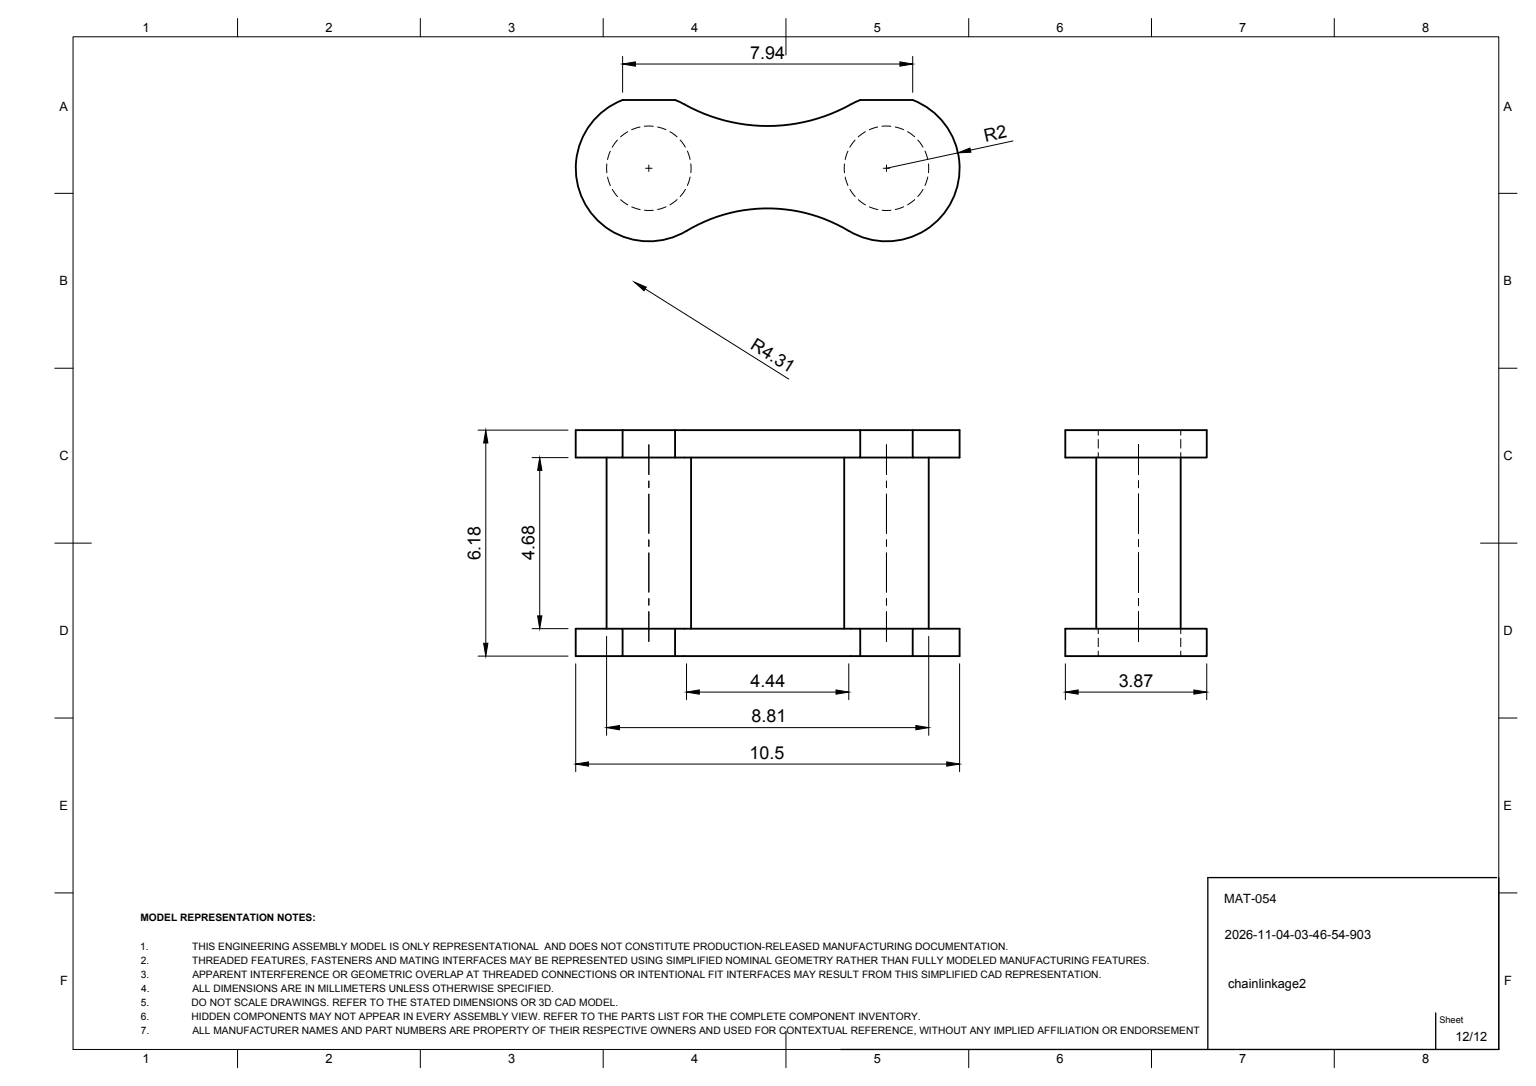
ISO-10303-21;
HEADER;
FILE_DESCRIPTION (('STEP AP214'),
    '1' );
FILE_NAME ('chainlinkage2.step',
    '2026-10-21T17:50:41',
    ( '' ),
    ( '' ),
    'SwSTEP 2.0',
    'SolidWorks 2026',
    '' );
FILE_SCHEMA (( 'AUTOMOTIVE_DESIGN' ));
ENDSEC;

DATA;
#33=CYLINDRICAL_SURFACE ( 'NONE', #30156, 1.999999999999999556 ) ;
#57=AXIS2_PLACEMENT_3D ( 'NONE', #27982, #32829, #17674 ) ;
#76=FACE_OUTER_BOUND ( 'NONE', #742, .T. ) ;
#123=DIRECTION ( 'NONE',  ( -0.000000000000000000, -0.000000000000000000, -1.000000000000000000 ) ) ;
#148=ORIENTED_EDGE ( 'NONE', *, *, #23576, .T. ) ;
#153=FACE_OUTER_BOUND ( 'NONE', #33687, .T. ) ;
#161=AXIS2_PLACEMENT_3D ( 'NONE', #27880, #20415, #25206 ) ;
#192=VERTEX_POINT ( 'NONE', #13936 ) ;
#226=CIRCLE ( 'NONE', #8162, 1.999999999999999112 ) ;
#270=ORIENTED_EDGE ( 'NONE', *, *, #32963, .T. ) ;
#279=CIRCLE ( 'NONE', #22435, 4.682234377621698584 ) ;
#283=CIRCLE ( 'NONE', #32662, 4.682234377621698584 ) ;
#306=DIRECTION ( 'NONE',  ( -0.000000000000000000, -0.000000000000000000, -1.000000000000000000 ) ) ;
#382=EDGE_CURVE ( 'NONE', #29286, #20322, #3767, .T. ) ;
#445=DIRECTION ( 'NONE',  ( 1.000000000000000000, 0.000000000000000000, 0.000000000000000000 ) ) ;
#472=CARTESIAN_POINT ( 'NONE',  ( -5.781867695661277118, -1.866624223957557893, -0.7500000000000000000 ) ) ;
#526=ORIENTED_EDGE ( 'NONE', *, *, #22218, .F. ) ;
#607=ORIENTED_EDGE ( 'NONE', *, *, #23373, .T. ) ;
#610=EDGE_CURVE ( 'NONE', #19346, #10620, #34542, .T. ) ;
#657=EDGE_CURVE ( 'NONE', #30105, #32001, #24381, .T. ) ;
#669=DIRECTION ( 'NONE',  ( -1.000000000000000000, 0.000000000000000000, 0.000000000000000000 ) ) ;
#680=ORIENTED_EDGE ( 'NONE', *, *, #6279, .T. ) ;
#740=CARTESIAN_POINT ( 'NONE',  ( -8.499999999999998224, 0.000000000000000000, 5.429999999999999716 ) ) ;
#742=EDGE_LOOP ( 'NONE', ( #25177, #23804, #31066, #16632 ) ) ;
#807=ORIENTED_EDGE ( 'NONE', *, *, #3982, .T. ) ;
#962=AXIS2_PLACEMENT_3D ( 'NONE', #16567, #5499, #19235 ) ;
#981=CARTESIAN_POINT ( 'NONE',  ( -0.9727285265192158192, -1.747512292859697114, 5.429999999999999716 ) ) ;
#994=ORIENTED_EDGE ( 'NONE', *, *, #20204, .T. ) ;
#1062=AXIS2_PLACEMENT_3D ( 'NONE', #28487, #22452, #19618 ) ;
#1071=CARTESIAN_POINT ( 'NONE',  ( -7.218132304338721994, -1.866624223957557893, -0.7500000000000000000 ) ) ;
#1096=AXIS2_PLACEMENT_3D ( 'NONE', #14859, #9508, #17884 ) ;
#1169=CARTESIAN_POINT ( 'NONE',  ( -0.7181323043387224381, -1.866624223957557893, 5.429999999999999716 ) ) ;
#1232=VECTOR ( 'NONE', #14059, 1000.000000000000000 ) ;
#1326=CARTESIAN_POINT ( 'NONE',  ( -6.500000000000000000, 0.000000000000000000, 4.679999999999999716 ) ) ;
#1403=ADVANCED_FACE ( 'NONE', ( #7003 ), #23561, .T. ) ;
#1433=CARTESIAN_POINT ( 'NONE',  ( -6.500000000000000000, 0.000000000000000000, -0.7500000000000000000 ) ) ;
#1457=DIRECTION ( 'NONE',  ( 1.000000000000000000, 0.000000000000000000, 0.000000000000000000 ) ) ;
#1552=ORIENTED_EDGE ( 'NONE', *, *, #6009, .F. ) ;
#1599=EDGE_CURVE ( 'NONE', #27420, #3383, #29381, .T. ) ;
#1635=EDGE_CURVE ( 'NONE', #15525, #19610, #9424, .T. ) ;
#1664=DIRECTION ( 'NONE',  ( 1.000000000000000000, 0.000000000000000000, -0.000000000000000000 ) ) ;
#1772=CARTESIAN_POINT ( 'NONE',  ( -5.527271473480783293, -1.747512292859696226, -0.7500000000000000000 ) ) ;
#1795=DIRECTION ( 'NONE',  ( -0.000000000000000000, -0.000000000000000000, 1.000000000000000000 ) ) ;
#1801=VERTEX_POINT ( 'NONE', #11106 ) ;
#1824=ORIENTED_EDGE ( 'NONE', *, *, #20677, .F. ) ;
#1889=EDGE_CURVE ( 'NONE', #30258, #28753, #22427, .T. ) ;
#1906=ORIENTED_EDGE ( 'NONE', *, *, #14574, .T. ) ;
#1963=DIRECTION ( 'NONE',  ( 0.000000000000000000, 0.000000000000000000, 1.000000000000000000 ) ) ;
#2042=ORIENTED_EDGE ( 'NONE', *, *, #610, .T. ) ;
#2140=FACE_OUTER_BOUND ( 'NONE', #7438, .T. ) ;
#2145=EDGE_CURVE ( 'NONE', #12065, #19610, #21352, .T. ) ;
#2200=DIRECTION ( 'NONE',  ( 0.000000000000000000, 0.000000000000000000, 1.000000000000000000 ) ) ;
#2218=DIRECTION ( 'NONE',  ( -0.000000000000000000, -0.000000000000000000, 1.000000000000000000 ) ) ;
#2279=CYLINDRICAL_SURFACE ( 'NONE', #5773, 4.306175033202026547 ) ;
#2373=CARTESIAN_POINT ( 'NONE',  ( -3.250000000000000000, -5.838643359331793015, 0.000000000000000000 ) ) ;
#2446=EDGE_LOOP ( 'NONE', ( #12551, #26713, #15573, #807 ) ) ;
#2510=CARTESIAN_POINT ( 'NONE',  ( -0.9727285265192158192, -1.747512292859697114, 5.429999999999999716 ) ) ;
#2547=EDGE_LOOP ( 'NONE', ( #27809, #20644, #34283, #22240 ) ) ;
#2562=EDGE_CURVE ( 'NONE', #24130, #18561, #30361, .T. ) ;
#2601=DIRECTION ( 'NONE',  ( -0.000000000000000000, -0.000000000000000000, 1.000000000000000000 ) ) ;
#2706=DIRECTION ( 'NONE',  ( 0.000000000000000000, 0.000000000000000000, 1.000000000000000000 ) ) ;
#2718=EDGE_CURVE ( 'NONE', #20895, #32553, #27626, .T. ) ;
#2738=LINE ( 'NONE', #10594, #16975 ) ;
#2747=CARTESIAN_POINT ( 'NONE',  ( -8.499999999999998224, 0.000000000000000000, 5.429999999999999716 ) ) ;
#2801=CARTESIAN_POINT ( 'NONE',  ( -5.781867695661277118, -1.866624223957557671, 0.000000000000000000 ) ) ;
#2898=AXIS2_PLACEMENT_3D ( 'NONE', #17177, #17360, #3961 ) ;
#2943=ORIENTED_EDGE ( 'NONE', *, *, #23576, .F. ) ;
#3000=LINE ( 'NONE', #33080, #33940 ) ;
#3027=EDGE_LOOP ( 'NONE', ( #24950, #28921 ) ) ;
#3202=EDGE_CURVE ( 'NONE', #20895, #30258, #14676, .T. ) ;
#3264=ORIENTED_EDGE ( 'NONE', *, *, #15668, .T. ) ;
#3331=CYLINDRICAL_SURFACE ( 'NONE', #18823, 1.999999999999999556 ) ;
#3383=VERTEX_POINT ( 'NONE', #7675 ) ;
#3421=EDGE_LOOP ( 'NONE', ( #14691, #9777, #5394, #24495 ) ) ;
#3565=FACE_OUTER_BOUND ( 'NONE', #34074, .T. ) ;
#3575=DIRECTION ( 'NONE',  ( -0.000000000000000000, -0.000000000000000000, 1.000000000000000000 ) ) ;
#3586=CARTESIAN_POINT ( 'NONE',  ( -6.500000000000000000, 0.000000000000000000, 5.429999999999999716 ) ) ;
#3600=DIRECTION ( 'NONE',  ( 0.000000000000000000, 0.000000000000000000, -1.000000000000000000 ) ) ;
#3637=EDGE_LOOP ( 'NONE', ( #26902, #13289, #29468, #6440 ) ) ;
#3645=AXIS2_PLACEMENT_3D ( 'NONE', #27958, #9269, #24755 ) ;
#3673=EDGE_LOOP ( 'NONE', ( #24652, #23698 ) ) ;
#3680=EDGE_CURVE ( 'NONE', #29286, #8432, #26053, .T. ) ;
#3707=LINE ( 'NONE', #11740, #27308 ) ;
#3708=ORIENTED_EDGE ( 'NONE', *, *, #1599, .F. ) ;
#3740=ORIENTED_EDGE ( 'NONE', *, *, #1599, .T. ) ;
#3752=AXIS2_PLACEMENT_3D ( 'NONE', #13925, #19628, #2706 ) ;
#3767=LINE ( 'NONE', #22120, #5990 ) ;
#3899=VECTOR ( 'NONE', #5620, 1000.000000000000000 ) ;
#3961=DIRECTION ( 'NONE',  ( -1.000000000000000000, 0.000000000000000000, 0.000000000000000000 ) ) ;
#3982=EDGE_CURVE ( 'NONE', #28753, #32553, #7816, .T. ) ;
#3987=ORIENTED_EDGE ( 'NONE', *, *, #33054, .F. ) ;
#4008=CIRCLE ( 'NONE', #57, 1.154999999999999805 ) ;
#4040=CARTESIAN_POINT ( 'NONE',  ( -6.500000000000000000, 0.000000000000000000, 5.429999999999999716 ) ) ;
#4043=DIRECTION ( 'NONE',  ( -0.000000000000000000, -0.000000000000000000, 1.000000000000000000 ) ) ;
#4060=DIRECTION ( 'NONE',  ( -1.000000000000000000, 0.000000000000000000, 0.000000000000000000 ) ) ;
#4081=DIRECTION ( 'NONE',  ( 0.000000000000000000, 0.000000000000000000, 1.000000000000000000 ) ) ;
#4084=ORIENTED_EDGE ( 'NONE', *, *, #2562, .F. ) ;
#4105=DIRECTION ( 'NONE',  ( -0.000000000000000000, -0.000000000000000000, -1.000000000000000000 ) ) ;
#4153=DIRECTION ( 'NONE',  ( -0.000000000000000000, -0.000000000000000000, 1.000000000000000000 ) ) ;
#4248=EDGE_LOOP ( 'NONE', ( #3740, #27735, #10056, #18991 ) ) ;
#4252=EDGE_CURVE ( 'NONE', #20322, #28753, #7368, .T. ) ;
#4270=ORIENTED_EDGE ( 'NONE', *, *, #32781, .T. ) ;
#4272=PLANE ( 'NONE',  #13542 ) ;
#4320=CARTESIAN_POINT ( 'NONE',  ( -1.625000000000000000, 2.702098422956710877, 4.679999999999999716 ) ) ;
#4327=CARTESIAN_POINT ( 'NONE',  ( -3.250000000000000000, 5.404196845913421754, -0.7500000000000000000 ) ) ;
#4356=ADVANCED_FACE ( 'NONE', ( #76 ), #10938, .T. ) ;
#4360=VERTEX_POINT ( 'NONE', #6274 ) ;
#4475=DIRECTION ( 'NONE',  ( -0.000000000000000000, -0.000000000000000000, -1.000000000000000000 ) ) ;
#4484=VECTOR ( 'NONE', #15412, 1000.000000000000000 ) ;
#4561=EDGE_CURVE ( 'NONE', #32547, #7170, #25532, .T. ) ;
#4648=CARTESIAN_POINT ( 'NONE',  ( -0.7181323043387224381, -1.866624223957557893, -0.7500000000000000000 ) ) ;
#4699=LINE ( 'NONE', #2747, #20213 ) ;
#4788=EDGE_CURVE ( 'NONE', #25489, #15525, #27437, .T. ) ;
#4841=APPLICATION_CONTEXT ( 'automotive_design' ) ;
#4877=CIRCLE ( 'NONE', #28201, 1.154999999999999805 ) ;
#4907=AXIS2_PLACEMENT_3D ( 'NONE', #20412, #12059, #23256 ) ;
#5009=LINE ( 'NONE', #24050, #23783 ) ;
#5104=CARTESIAN_POINT ( 'NONE',  ( -5.781867695661277118, -1.866624223957557671, 4.679999999999999716 ) ) ;
#5132=DIRECTION ( 'NONE',  ( 1.000000000000000000, 0.000000000000000000, 0.000000000000000000 ) ) ;
#5180=FACE_OUTER_BOUND ( 'NONE', #20182, .T. ) ;
#5206=EDGE_CURVE ( 'NONE', #24311, #10245, #32875, .T. ) ;
#5210=ORIENTED_EDGE ( 'NONE', *, *, #34210, .F. ) ;
#5394=ORIENTED_EDGE ( 'NONE', *, *, #14375, .T. ) ;
#5415=DIRECTION ( 'NONE',  ( 1.000000000000000000, 0.000000000000000000, 0.000000000000000000 ) ) ;
#5431=ORIENTED_EDGE ( 'NONE', *, *, #19622, .T. ) ;
#5455=LINE ( 'NONE', #13653, #3899 ) ;
#5456=ORIENTED_EDGE ( 'NONE', *, *, #15677, .F. ) ;
#5499=DIRECTION ( 'NONE',  ( 0.000000000000000000, 0.000000000000000000, -1.000000000000000000 ) ) ;
#5531=DIRECTION ( 'NONE',  ( -0.000000000000000000, -0.000000000000000000, -1.000000000000000000 ) ) ;
#5620=DIRECTION ( 'NONE',  ( 1.000000000000000000, -0.000000000000000000, -0.000000000000000000 ) ) ;
#5648=VECTOR ( 'NONE', #5531, 1000.000000000000000 ) ;
#5753=CYLINDRICAL_SURFACE ( 'NONE', #12901, 1.999999999999999556 ) ;
#5773=AXIS2_PLACEMENT_3D ( 'NONE', #10296, #13502, #24337 ) ;
#5812=ADVANCED_FACE ( 'NONE', ( #3565 ), #22273, .T. ) ;
#5894=( NAMED_UNIT ( * ) SI_UNIT ( $, .STERADIAN. ) SOLID_ANGLE_UNIT ( ) );
#5905=CIRCLE ( 'NONE', #29220, 1.155000000000000027 ) ;
#5962=CARTESIAN_POINT ( 'NONE',  ( -7.218132304338721994, -1.866624223957557893, 5.429999999999999716 ) ) ;
#5972=DIRECTION ( 'NONE',  ( -1.000000000000000000, 0.000000000000000000, 0.000000000000000000 ) ) ;
#5990=VECTOR ( 'NONE', #8937, 1000.000000000000000 ) ;
#6009=EDGE_CURVE ( 'NONE', #10891, #18561, #14477, .T. ) ;
#6062=ORIENTED_EDGE ( 'NONE', *, *, #32625, .F. ) ;
#6080=EDGE_CURVE ( 'NONE', #14482, #29522, #13328, .T. ) ;
#6147=CARTESIAN_POINT ( 'NONE',  ( 0.7181323043387221050, -1.866624223957557893, -0.7500000000000000000 ) ) ;
#6183=ORIENTED_EDGE ( 'NONE', *, *, #382, .F. ) ;
#6198=ORIENTED_EDGE ( 'NONE', *, *, #657, .F. ) ;
#6223=CARTESIAN_POINT ( 'NONE',  ( 0.000000000000000000, 0.000000000000000000, -0.7500000000000000000 ) ) ;
#6274=CARTESIAN_POINT ( 'NONE',  ( -5.781867695661277118, -1.866624223957557893, 5.429999999999999716 ) ) ;
#6276=CARTESIAN_POINT ( 'NONE',  ( 2.630124765083918348, -1.866624223957557893, 5.429999999999999716 ) ) ;
#6279=EDGE_CURVE ( 'NONE', #8432, #10891, #283, .T. ) ;
#6364=ORIENTED_EDGE ( 'NONE', *, *, #22218, .T. ) ;
#6440=ORIENTED_EDGE ( 'NONE', *, *, #12810, .T. ) ;
#6484=ORIENTED_EDGE ( 'NONE', *, *, #28737, .F. ) ;
#6499=ORIENTED_EDGE ( 'NONE', *, *, #23373, .F. ) ;
#6540=PLANE ( 'NONE',  #23252 ) ;
#6625=AXIS2_PLACEMENT_3D ( 'NONE', #7346, #10210, #28729 ) ;
#6650=ADVANCED_FACE ( 'NONE', ( #32164 ), #13134, .T. ) ;
#6750=AXIS2_PLACEMENT_3D ( 'NONE', #22899, #25556, #33751 ) ;
#6774=DIRECTION ( 'NONE',  ( 0.000000000000000000, 1.000000000000000000, -0.000000000000000000 ) ) ;
#6790=( LENGTH_UNIT ( ) NAMED_UNIT ( * ) SI_UNIT ( .MILLI., .METRE. ) );
#6808=DIRECTION ( 'NONE',  ( -1.000000000000000000, 0.000000000000000000, 0.000000000000000000 ) ) ;
#6821=DIRECTION ( 'NONE',  ( -0.000000000000000000, -0.000000000000000000, -1.000000000000000000 ) ) ;
#6836=VERTEX_POINT ( 'NONE', #33564 ) ;
#6850=DIRECTION ( 'NONE',  ( 1.000000000000000000, 0.000000000000000000, 0.000000000000000000 ) ) ;
#6866=CARTESIAN_POINT ( 'NONE',  ( -3.250000000000000000, 5.404196845913421754, 5.429999999999999716 ) ) ;
#6941=CARTESIAN_POINT ( 'NONE',  ( 2.630124765083918348, -1.866624223957557893, 5.429999999999999716 ) ) ;
#6960=( NAMED_UNIT ( * ) SI_UNIT ( $, .STERADIAN. ) SOLID_ANGLE_UNIT ( ) );
#7003=FACE_OUTER_BOUND ( 'NONE', #3637, .T. ) ;
#7012=DIRECTION ( 'NONE',  ( 1.000000000000000000, 0.000000000000000000, 0.000000000000000000 ) ) ;
#7051=VECTOR ( 'NONE', #1795, 1000.000000000000000 ) ;
#7067=CARTESIAN_POINT ( 'NONE',  ( -6.500000000000000000, 0.000000000000000000, 0.000000000000000000 ) ) ;
#7073=VERTEX_POINT ( 'NONE', #7914 ) ;
#7107=CARTESIAN_POINT ( 'NONE',  ( -6.500000000000000000, 0.000000000000000000, 5.429999999999999716 ) ) ;
#7145=DIRECTION ( 'NONE',  ( 0.000000000000000000, 0.000000000000000000, 1.000000000000000000 ) ) ;
#7170=VERTEX_POINT ( 'NONE', #22325 ) ;
#7205=CARTESIAN_POINT ( 'NONE',  ( -5.527271473480783293, -1.747512292859696226, 5.429999999999999716 ) ) ;
#7230=CARTESIAN_POINT ( 'NONE',  ( -1.030735741678193484, 1.713938105891546826, 0.000000000000000000 ) ) ;
#7325=DIRECTION ( 'NONE',  ( 0.000000000000000000, 0.000000000000000000, 1.000000000000000000 ) ) ;
#7346=CARTESIAN_POINT ( 'NONE',  ( 0.000000000000000000, 0.000000000000000000, 4.679999999999999716 ) ) ;
#7368=LINE ( 'NONE', #34983, #4484 ) ;
#7438=EDGE_LOOP ( 'NONE', ( #13903, #20764, #6198, #1824 ) ) ;
#7472=DIRECTION ( 'NONE',  ( 0.000000000000000000, 0.000000000000000000, 1.000000000000000000 ) ) ;
#7500=EDGE_LOOP ( 'NONE', ( #17353, #22619, #28907, #19252 ) ) ;
#7618=ADVANCED_FACE ( 'NONE', ( #16787 ), #21583, .F. ) ;
#7628=DIRECTION ( 'NONE',  ( -0.000000000000000000, -0.000000000000000000, -1.000000000000000000 ) ) ;
#7675=CARTESIAN_POINT ( 'NONE',  ( -5.527271473480783293, -1.747512292859696226, 0.000000000000000000 ) ) ;
#7677=ORIENTED_EDGE ( 'NONE', *, *, #1635, .T. ) ;
#7816=LINE ( 'NONE', #6147, #34613 ) ;
#7914=CARTESIAN_POINT ( 'NONE',  ( -5.469264258321805627, 1.713938105891546382, -0.7500000000000000000 ) ) ;
#7930=DIRECTION ( 'NONE',  ( 0.000000000000000000, 0.000000000000000000, 1.000000000000000000 ) ) ;
#7953=CARTESIAN_POINT ( 'NONE',  ( -5.781867695661277118, -1.866624223957557893, 5.429999999999999716 ) ) ;
#7982=AXIS2_PLACEMENT_3D ( 'NONE', #19006, #123, #5972 ) ;
#8095=ORIENTED_EDGE ( 'NONE', *, *, #9484, .F. ) ;
#8124=( GEOMETRIC_REPRESENTATION_CONTEXT ( 3 ) GLOBAL_UNCERTAINTY_ASSIGNED_CONTEXT ( ( #10711 ) ) GLOBAL_UNIT_ASSIGNED_CONTEXT ( ( #6790, #17854, #6960 ) ) REPRESENTATION_CONTEXT ( 'NONE', 'WORKASPACE' ) );
#8162=AXIS2_PLACEMENT_3D ( 'NONE', #16370, #27200, #18690 ) ;
#8188=ADVANCED_FACE ( 'NONE', ( #31428 ), #12407, .T. ) ;
#8209=ORIENTED_EDGE ( 'NONE', *, *, #20677, .T. ) ;
#8237=EDGE_CURVE ( 'NONE', #25058, #192, #14735, .T. ) ;
#8298=DIRECTION ( 'NONE',  ( -1.000000000000000000, 0.000000000000000000, 0.000000000000000000 ) ) ;
#8328=VECTOR ( 'NONE', #23417, 1000.000000000000000 ) ;
#8350=EDGE_CURVE ( 'NONE', #29522, #33375, #4699, .T. ) ;
#8432=VERTEX_POINT ( 'NONE', #21094 ) ;
#8444=ADVANCED_FACE ( 'NONE', ( #19148 ), #5753, .T. ) ;
#8460=ORIENTED_EDGE ( 'NONE', *, *, #17006, .F. ) ;
#8549=ORIENTED_EDGE ( 'NONE', *, *, #14574, .F. ) ;
#8594=VECTOR ( 'NONE', #28010, 1000.000000000000000 ) ;
#8684=FACE_OUTER_BOUND ( 'NONE', #19828, .T. ) ;
#8792=CIRCLE ( 'NONE', #25839, 1.999999999999999112 ) ;
#8812=FACE_BOUND ( 'NONE', #3673, .T. ) ;
#8822=DIRECTION ( 'NONE',  ( 0.000000000000000000, 0.000000000000000000, -1.000000000000000000 ) ) ;
#8913=DIRECTION ( 'NONE',  ( 1.000000000000000000, 0.000000000000000000, 0.000000000000000000 ) ) ;
#8937=DIRECTION ( 'NONE',  ( -0.000000000000000000, -0.000000000000000000, 1.000000000000000000 ) ) ;
#8941=CARTESIAN_POINT ( 'NONE',  ( -1.155000000000000027, 0.000000000000000000, 4.679999999999999716 ) ) ;
#8944=LINE ( 'NONE', #19816, #15535 ) ;
#9132=CARTESIAN_POINT ( 'NONE',  ( -6.500000000000000000, 0.000000000000000000, 4.679999999999999716 ) ) ;
#9140=AXIS2_PLACEMENT_3D ( 'NONE', #25229, #13124, #10266 ) ;
#9166=VERTEX_POINT ( 'NONE', #13020 ) ;
#9191=ORIENTED_EDGE ( 'NONE', *, *, #17768, .T. ) ;
#9269=DIRECTION ( 'NONE',  ( -0.000000000000000000, -0.000000000000000000, 1.000000000000000000 ) ) ;
#9292=EDGE_CURVE ( 'NONE', #26696, #10620, #16968, .T. ) ;
#9307=CARTESIAN_POINT ( 'NONE',  ( 0.000000000000000000, 0.000000000000000000, 0.000000000000000000 ) ) ;
#9356=AXIS2_PLACEMENT_3D ( 'NONE', #7107, #4081, #14977 ) ;
#9424=CIRCLE ( 'NONE', #32699, 1.999999999999999556 ) ;
#9484=EDGE_CURVE ( 'NONE', #15525, #19346, #14950, .T. ) ;
#9508=DIRECTION ( 'NONE',  ( -0.000000000000000000, -0.000000000000000000, -1.000000000000000000 ) ) ;
#9509=EDGE_LOOP ( 'NONE', ( #3264, #2042, #19117, #17931 ) ) ;
#9514=DIRECTION ( 'NONE',  ( 0.000000000000000000, 0.000000000000000000, 1.000000000000000000 ) ) ;
#9533=EDGE_CURVE ( 'NONE', #31862, #9166, #17099, .T. ) ;
#9557=ORIENTED_EDGE ( 'NONE', *, *, #17768, .F. ) ;
#9777=ORIENTED_EDGE ( 'NONE', *, *, #28737, .T. ) ;
#10056=ORIENTED_EDGE ( 'NONE', *, *, #6279, .F. ) ;
#10119=ADVANCED_FACE ( 'NONE', ( #153 ), #26678, .T. ) ;
#10166=ADVANCED_FACE ( 'NONE', ( #8684 ), #6540, .F. ) ;
#10191=CARTESIAN_POINT ( 'NONE',  ( -6.500000000000000000, 0.000000000000000000, 5.429999999999999716 ) ) ;
#10210=DIRECTION ( 'NONE',  ( -0.000000000000000000, -0.000000000000000000, -1.000000000000000000 ) ) ;
#10245=VERTEX_POINT ( 'NONE', #7230 ) ;
#10266=DIRECTION ( 'NONE',  ( -1.000000000000000000, 0.000000000000000000, 0.000000000000000000 ) ) ;
#10296=CARTESIAN_POINT ( 'NONE',  ( -3.250000000000000000, 5.404196845913421754, -0.7500000000000000000 ) ) ;
#10368=CARTESIAN_POINT ( 'NONE',  ( 1.999999999999999556, 0.000000000000000000, -0.7500000000000000000 ) ) ;
#10410=MECHANICAL_DESIGN_GEOMETRIC_PRESENTATION_REPRESENTATION('',(#34291),#14976);
#10424=CARTESIAN_POINT ( 'NONE',  ( -7.654999999999999361, 1.414467053015192657E-16, 0.000000000000000000 ) ) ;
#10486=EDGE_CURVE ( 'NONE', #32001, #1801, #22005, .T. ) ;
#10493=CARTESIAN_POINT ( 'NONE',  ( -6.500000000000000000, 0.000000000000000000, -0.7500000000000000000 ) ) ;
#10594=CARTESIAN_POINT ( 'NONE',  ( -5.344999999999999751, 0.000000000000000000, -0.7520000000000001128 ) ) ;
#10601=ORIENTED_EDGE ( 'NONE', *, *, #4788, .F. ) ;
#10603=DIRECTION ( 'NONE',  ( -0.000000000000000000, -0.000000000000000000, -1.000000000000000000 ) ) ;
#10620=VERTEX_POINT ( 'NONE', #1169 ) ;
#10656=ORIENTED_EDGE ( 'NONE', *, *, #15964, .F. ) ;
#10662=ORIENTED_EDGE ( 'NONE', *, *, #6080, .F. ) ;
#10700=EDGE_CURVE ( 'NONE', #7073, #24311, #14887, .T. ) ;
#10709=ORIENTED_EDGE ( 'NONE', *, *, #8350, .F. ) ;
#10711=UNCERTAINTY_MEASURE_WITH_UNIT (LENGTH_MEASURE( 1.000000000000000082E-05 ), #6790, 'distance_accuracy_value', 'NONE');
#10748=AXIS2_PLACEMENT_3D ( 'NONE', #10493, #21351, #22219 ) ;
#10774=EDGE_CURVE ( 'NONE', #26696, #12145, #24396, .T. ) ;
#10791=DIRECTION ( 'NONE',  ( 1.000000000000000000, 0.000000000000000000, 0.000000000000000000 ) ) ;
#10825=ADVANCED_FACE ( 'NONE', ( #14974 ), #32408, .T. ) ;
#10826=CARTESIAN_POINT ( 'NONE',  ( -4.875000000000000000, 2.702098422956710877, 0.000000000000000000 ) ) ;
#10854=LINE ( 'NONE', #32734, #1232 ) ;
#10867=DIRECTION ( 'NONE',  ( -1.000000000000000000, 0.000000000000000000, 0.000000000000000000 ) ) ;
#10887=DIRECTION ( 'NONE',  ( -0.000000000000000000, -0.000000000000000000, -1.000000000000000000 ) ) ;
#10891=VERTEX_POINT ( 'NONE', #1772 ) ;
#10938=CYLINDRICAL_SURFACE ( 'NONE', #15316, 1.999999999999999112 ) ;
#10944=DIRECTION ( 'NONE',  ( -0.000000000000000000, -0.000000000000000000, 1.000000000000000000 ) ) ;
#10974=VERTEX_POINT ( 'NONE', #33997 ) ;
#11099=CLOSED_SHELL ( 'NONE', ( #21470, #4356, #8444, #6650, #25183, #8188, #29310, #19441, #1403, #34762, #10825, #23574, #10119, #21762, #26582, #23268, #15805, #23565, #13258, #15277, #25660, #5812, #21609, #13668, #10166, #7618 ) ) ;
#11106=CARTESIAN_POINT ( 'NONE',  ( -7.218132304338721994, -1.866624223957557893, 5.429999999999999716 ) ) ;
#11108=ORIENTED_EDGE ( 'NONE', *, *, #32781, .F. ) ;
#11136=EDGE_CURVE ( 'NONE', #25489, #12065, #16989, .T. ) ;
#11168=CYLINDRICAL_SURFACE ( 'NONE', #7982, 4.306175033202026547 ) ;
#11202=PRODUCT ( 'chainlinkage2', 'chainlinkage2', '', ( #13725 ) ) ;
#11219=VECTOR ( 'NONE', #8822, 1000.000000000000000 ) ;
#11416=EDGE_LOOP ( 'NONE', ( #10709, #10662, #6364, #24149 ) ) ;
#11435=CARTESIAN_POINT ( 'NONE',  ( 0.7181323043387224381, -1.866624223957557893, -0.7500000000000000000 ) ) ;
#11453=CARTESIAN_POINT ( 'NONE',  ( -5.344999999999999751, 0.000000000000000000, 4.679999999999999716 ) ) ;
#11454=AXIS2_PLACEMENT_3D ( 'NONE', #31541, #7145, #25676 ) ;
#11481=CARTESIAN_POINT ( 'NONE',  ( 0.7181323043387224381, -1.866624223957557893, 5.429999999999999716 ) ) ;
#11525=ORIENTED_EDGE ( 'NONE', *, *, #3680, .T. ) ;
#11634=VECTOR ( 'NONE', #7628, 1000.000000000000000 ) ;
#11740=CARTESIAN_POINT ( 'NONE',  ( -7.218132304338721994, -1.866624223957557893, -0.7500000000000000000 ) ) ;
#11795=DIRECTION ( 'NONE',  ( 1.000000000000000000, 0.000000000000000000, 0.000000000000000000 ) ) ;
#11865=DIRECTION ( 'NONE',  ( -0.000000000000000000, -0.000000000000000000, -1.000000000000000000 ) ) ;
#11869=EDGE_CURVE ( 'NONE', #30622, #18057, #2738, .T. ) ;
#11921=DIRECTION ( 'NONE',  ( -1.000000000000000000, 0.000000000000000000, 0.000000000000000000 ) ) ;
#11987=AXIS2_PLACEMENT_3D ( 'NONE', #6866, #31437, #23266 ) ;
#12059=DIRECTION ( 'NONE',  ( -0.000000000000000000, -0.000000000000000000, 1.000000000000000000 ) ) ;
#12065=VERTEX_POINT ( 'NONE', #23537 ) ;
#12092=CARTESIAN_POINT ( 'NONE',  ( 0.7181323043387224381, -1.866624223957557671, 4.679999999999999716 ) ) ;
#12127=CARTESIAN_POINT ( 'NONE',  ( -1.155000000000000027, 0.000000000000000000, 0.000000000000000000 ) ) ;
#12145=VERTEX_POINT ( 'NONE', #15019 ) ;
#12180=DIRECTION ( 'NONE',  ( -0.000000000000000000, -0.000000000000000000, -1.000000000000000000 ) ) ;
#12182=CARTESIAN_POINT ( 'NONE',  ( -6.500000000000000000, 0.000000000000000000, 5.429999999999999716 ) ) ;
#12220=CARTESIAN_POINT ( 'NONE',  ( -5.469264258321805627, 1.713938105891546382, -0.7500000000000000000 ) ) ;
#12222=DIRECTION ( 'NONE',  ( 0.000000000000000000, 0.000000000000000000, -1.000000000000000000 ) ) ;
#12304=EDGE_CURVE ( 'NONE', #8432, #27420, #5009, .T. ) ;
#12346=EDGE_LOOP ( 'NONE', ( #32721, #16598, #34085, #28075 ) ) ;
#12347=DIRECTION ( 'NONE',  ( -1.000000000000000000, 0.000000000000000000, 0.000000000000000000 ) ) ;
#12407=CYLINDRICAL_SURFACE ( 'NONE', #4907, 1.999999999999999112 ) ;
#12426=EDGE_CURVE ( 'NONE', #23952, #7073, #34016, .T. ) ;
#12508=DIRECTION ( 'NONE',  ( 0.000000000000000000, 1.000000000000000000, -0.000000000000000000 ) ) ;
#12551=ORIENTED_EDGE ( 'NONE', *, *, #2718, .F. ) ;
#12553=CARTESIAN_POINT ( 'NONE',  ( -3.250000000000000000, -5.838643359331793015, 5.429999999999999716 ) ) ;
#12584=ORIENTED_EDGE ( 'NONE', *, *, #15594, .F. ) ;
#12623=VECTOR ( 'NONE', #26656, 1000.000000000000000 ) ;
#12670=EDGE_CURVE ( 'NONE', #23952, #18561, #5455, .T. ) ;
#12810=EDGE_CURVE ( 'NONE', #14097, #6836, #17585, .T. ) ;
#12849=DIRECTION ( 'NONE',  ( 1.000000000000000000, 0.000000000000000000, 0.000000000000000000 ) ) ;
#12865=EDGE_LOOP ( 'NONE', ( #29599, #18345, #9557, #34184 ) ) ;
#12877=DIRECTION ( 'NONE',  ( 0.000000000000000000, 0.000000000000000000, 1.000000000000000000 ) ) ;
#12899=DIRECTION ( 'NONE',  ( -1.000000000000000000, 0.000000000000000000, 0.000000000000000000 ) ) ;
#12901=AXIS2_PLACEMENT_3D ( 'NONE', #30151, #10944, #445 ) ;
#13020=CARTESIAN_POINT ( 'NONE',  ( -7.654999999999999361, 1.414467053015192657E-16, 4.679999999999999716 ) ) ;
#13060=PLANE ( 'NONE',  #20095 ) ;
#13073=DIRECTION ( 'NONE',  ( 1.000000000000000000, 0.000000000000000000, 0.000000000000000000 ) ) ;
#13124=DIRECTION ( 'NONE',  ( 0.000000000000000000, 0.000000000000000000, -1.000000000000000000 ) ) ;
#13134=CYLINDRICAL_SURFACE ( 'NONE', #26444, 1.155000000000000027 ) ;
#13254=DIRECTION ( 'NONE',  ( 1.000000000000000000, 0.000000000000000000, 0.000000000000000000 ) ) ;
#13258=ADVANCED_FACE ( 'NONE', ( #15376 ), #20198, .F. ) ;
#13289=ORIENTED_EDGE ( 'NONE', *, *, #4561, .F. ) ;
#13328=CIRCLE ( 'NONE', #9356, 1.999999999999999112 ) ;
#13374=CARTESIAN_POINT ( 'NONE',  ( -0.9727285265192152641, -1.747512292859696670, 0.000000000000000000 ) ) ;
#13418=AXIS2_PLACEMENT_3D ( 'NONE', #23360, #28185, #34219 ) ;
#13502=DIRECTION ( 'NONE',  ( -0.000000000000000000, -0.000000000000000000, 1.000000000000000000 ) ) ;
#13537=CARTESIAN_POINT ( 'NONE',  ( 0.000000000000000000, 0.000000000000000000, 5.429999999999999716 ) ) ;
#13542=AXIS2_PLACEMENT_3D ( 'NONE', #6941, #6774, #1963 ) ;
#13571=CARTESIAN_POINT ( 'NONE',  ( 0.7181323043387221050, -1.866624223957557893, 5.429999999999999716 ) ) ;
#13645=ORIENTED_EDGE ( 'NONE', *, *, #19386, .F. ) ;
#13653=CARTESIAN_POINT ( 'NONE',  ( 2.630124765083918348, -1.866624223957557893, -0.7500000000000000000 ) ) ;
#13668=ADVANCED_FACE ( 'NONE', ( #31360 ), #31532, .F. ) ;
#13707=DIRECTION ( 'NONE',  ( 0.000000000000000000, 0.000000000000000000, 1.000000000000000000 ) ) ;
#13715=CIRCLE ( 'NONE', #2898, 1.154999999999999805 ) ;
#13725=PRODUCT_CONTEXT ( 'NONE', #29182, 'mechanical' ) ;
#13903=ORIENTED_EDGE ( 'NONE', *, *, #20204, .F. ) ;
#13925=CARTESIAN_POINT ( 'NONE',  ( 2.630124765083918348, -1.866624223957557893, 5.429999999999999716 ) ) ;
#13936=CARTESIAN_POINT ( 'NONE',  ( -5.527271473480783293, -1.747512292859696226, 4.679999999999999716 ) ) ;
#13954=EDGE_LOOP ( 'NONE', ( #27650, #15530, #8095, #10601 ) ) ;
#14059=DIRECTION ( 'NONE',  ( -0.000000000000000000, -0.000000000000000000, -1.000000000000000000 ) ) ;
#14097=VERTEX_POINT ( 'NONE', #12127 ) ;
#14177=CARTESIAN_POINT ( 'NONE',  ( 2.630124765083918348, -1.866624223957557893, 5.429999999999999716 ) ) ;
#14182=VECTOR ( 'NONE', #17038, 1000.000000000000000 ) ;
#14209=CARTESIAN_POINT ( 'NONE',  ( 0.000000000000000000, 0.000000000000000000, 5.429999999999999716 ) ) ;
#14288=ORIENTED_EDGE ( 'NONE', *, *, #6009, .T. ) ;
#14375=EDGE_CURVE ( 'NONE', #22709, #24311, #34699, .T. ) ;
#14427=ORIENTED_EDGE ( 'NONE', *, *, #34210, .T. ) ;
#14450=CARTESIAN_POINT ( 'NONE',  ( -5.781867695661277118, -1.866624223957557893, -0.7500000000000000000 ) ) ;
#14469=LINE ( 'NONE', #22472, #16180 ) ;
#14477=CIRCLE ( 'NONE', #21840, 1.999999999999999112 ) ;
#14482=VERTEX_POINT ( 'NONE', #28616 ) ;
#14489=ORIENTED_EDGE ( 'NONE', *, *, #11869, .T. ) ;
#14574=EDGE_CURVE ( 'NONE', #30622, #31862, #21053, .T. ) ;
#14595=CARTESIAN_POINT ( 'NONE',  ( -0.7181323043387224381, -1.866624223957557671, 0.000000000000000000 ) ) ;
#14611=CARTESIAN_POINT ( 'NONE',  ( -7.654999999999999361, 1.414467053015192657E-16, -0.7520000000000001128 ) ) ;
#14657=DIRECTION ( 'NONE',  ( -0.000000000000000000, -0.000000000000000000, 1.000000000000000000 ) ) ;
#14676=LINE ( 'NONE', #22842, #22633 ) ;
#14691=ORIENTED_EDGE ( 'NONE', *, *, #12426, .F. ) ;
#14735=LINE ( 'NONE', #7205, #8328 ) ;
#14777=EDGE_CURVE ( 'NONE', #10245, #30258, #30763, .T. ) ;
#14784=AXIS2_PLACEMENT_3D ( 'NONE', #14177, #12508, #33198 ) ;
#14804=ORIENTED_EDGE ( 'NONE', *, *, #33054, .T. ) ;
#14822=CYLINDRICAL_SURFACE ( 'NONE', #19963, 4.682234377621698584 ) ;
#14837=ORIENTED_EDGE ( 'NONE', *, *, #11869, .F. ) ;
#14859=CARTESIAN_POINT ( 'NONE',  ( -3.250000000000000000, -5.838643359331793015, 5.429999999999999716 ) ) ;
#14887=LINE ( 'NONE', #12220, #22698 ) ;
#14890=DIRECTION ( 'NONE',  ( -1.000000000000000000, 0.000000000000000000, 0.000000000000000000 ) ) ;
#14905=FACE_OUTER_BOUND ( 'NONE', #7500, .T. ) ;
#14933=PRODUCT_DEFINITION_SHAPE ( 'NONE', 'NONE',  #21422 ) ;
#14938=CARTESIAN_POINT ( 'NONE',  ( 0.7181323043387224381, -1.866624223957557671, 0.000000000000000000 ) ) ;
#14950=LINE ( 'NONE', #22953, #32273 ) ;
#14974=FACE_OUTER_BOUND ( 'NONE', #12346, .T. ) ;
#14976=( GEOMETRIC_REPRESENTATION_CONTEXT ( 3 ) GLOBAL_UNCERTAINTY_ASSIGNED_CONTEXT ( ( #17148 ) ) GLOBAL_UNIT_ASSIGNED_CONTEXT ( ( #21935, #30293, #5894 ) ) REPRESENTATION_CONTEXT ( 'NONE', 'WORKASPACE' ) );
#14977=DIRECTION ( 'NONE',  ( 1.000000000000000000, 0.000000000000000000, 0.000000000000000000 ) ) ;
#15016=ORIENTED_EDGE ( 'NONE', *, *, #30130, .F. ) ;
#15017=ORIENTED_EDGE ( 'NONE', *, *, #11136, .F. ) ;
#15019=CARTESIAN_POINT ( 'NONE',  ( -0.9727285265192158192, -1.747512292859697114, 4.679999999999999716 ) ) ;
#15201=ORIENTED_EDGE ( 'NONE', *, *, #657, .T. ) ;
#15206=DIRECTION ( 'NONE',  ( 0.000000000000000000, 0.000000000000000000, 1.000000000000000000 ) ) ;
#15277=ADVANCED_FACE ( 'NONE', ( #20517 ), #20697, .T. ) ;
#15316=AXIS2_PLACEMENT_3D ( 'NONE', #12182, #20523, #6808 ) ;
#15357=EDGE_LOOP ( 'NONE', ( #12584, #8209, #4270, #23675 ) ) ;
#15376=FACE_OUTER_BOUND ( 'NONE', #12865, .T. ) ;
#15395=DIRECTION ( 'NONE',  ( 0.000000000000000000, -0.000000000000000000, 1.000000000000000000 ) ) ;
#15412=DIRECTION ( 'NONE',  ( 1.000000000000000000, 0.000000000000000000, 0.000000000000000000 ) ) ;
#15420=CIRCLE ( 'NONE', #11987, 4.306175033202026547 ) ;
#15525=VERTEX_POINT ( 'NONE', #12092 ) ;
#15530=ORIENTED_EDGE ( 'NONE', *, *, #610, .F. ) ;
#15535=VECTOR ( 'NONE', #22125, 1000.000000000000000 ) ;
#15573=ORIENTED_EDGE ( 'NONE', *, *, #1889, .T. ) ;
#15594=EDGE_CURVE ( 'NONE', #4360, #25058, #30200, .T. ) ;
#15595=AXIS2_PLACEMENT_3D ( 'NONE', #9307, #3600, #23480 ) ;
#15668=EDGE_CURVE ( 'NONE', #12145, #19346, #34212, .T. ) ;
#15677=EDGE_CURVE ( 'NONE', #3383, #24130, #18886, .T. ) ;
#15729=CARTESIAN_POINT ( 'NONE',  ( 0.000000000000000000, 0.000000000000000000, 5.429999999999999716 ) ) ;
#15738=FACE_BOUND ( 'NONE', #3027, .T. ) ;
#15767=SHAPE_REPRESENTATION ( 'chainlinkage2', ( #28566 ), #8124 ) ;
#15803=ORIENTED_EDGE ( 'NONE', *, *, #6080, .T. ) ;
#15805=ADVANCED_FACE ( 'NONE', ( #27169 ), #11168, .F. ) ;
#15812=ORIENTED_EDGE ( 'NONE', *, *, #12670, .F. ) ;
#15820=DIRECTION ( 'NONE',  ( -1.000000000000000000, 0.000000000000000000, 0.000000000000000000 ) ) ;
#15964=EDGE_CURVE ( 'NONE', #19610, #22312, #25029, .T. ) ;
#15997=ORIENTED_EDGE ( 'NONE', *, *, #3982, .F. ) ;
#16037=PLANE ( 'NONE',  #962 ) ;
#16130=CARTESIAN_POINT ( 'NONE',  ( -6.500000000000000000, 0.000000000000000000, 4.679999999999999716 ) ) ;
#16131=ORIENTED_EDGE ( 'NONE', *, *, #15668, .F. ) ;
#16180=VECTOR ( 'NONE', #16798, 1000.000000000000000 ) ;
#16212=DIRECTION ( 'NONE',  ( 1.000000000000000000, -0.000000000000000000, -0.000000000000000000 ) ) ;
#16370=CARTESIAN_POINT ( 'NONE',  ( -6.500000000000000000, 0.000000000000000000, 4.679999999999999716 ) ) ;
#16383=EDGE_CURVE ( 'NONE', #31862, #30622, #13715, .T. ) ;
#16488=EDGE_CURVE ( 'NONE', #10620, #25489, #30686, .T. ) ;
#16567=CARTESIAN_POINT ( 'NONE',  ( -4.875000000000000000, 2.702098422956710877, -0.7500000000000000000 ) ) ;
#16581=AXIS2_PLACEMENT_3D ( 'NONE', #4040, #17266, #28622 ) ;
#16598=ORIENTED_EDGE ( 'NONE', *, *, #32963, .F. ) ;
#16632=ORIENTED_EDGE ( 'NONE', *, *, #10486, .T. ) ;
#16633=EDGE_LOOP ( 'NONE', ( #15812, #24955, #26626, #270, #27986, #3987, #11525, #680, #14288 ) ) ;
#16731=CARTESIAN_POINT ( 'NONE',  ( -3.250000000000000000, -5.838643359331793015, -0.7500000000000000000 ) ) ;
#16756=CIRCLE ( 'NONE', #33791, 4.682234377621698584 ) ;
#16787=FACE_OUTER_BOUND ( 'NONE', #23195, .T. ) ;
#16798=DIRECTION ( 'NONE',  ( 1.000000000000000000, -0.000000000000000000, -0.000000000000000000 ) ) ;
#16968=CIRCLE ( 'NONE', #30415, 1.999999999999999556 ) ;
#16975=VECTOR ( 'NONE', #2218, 1000.000000000000000 ) ;
#16989=CIRCLE ( 'NONE', #17558, 1.999999999999999556 ) ;
#16998=DIRECTION ( 'NONE',  ( -0.000000000000000000, -0.000000000000000000, 1.000000000000000000 ) ) ;
#17006=EDGE_CURVE ( 'NONE', #33375, #32001, #226, .T. ) ;
#17038=DIRECTION ( 'NONE',  ( 0.000000000000000000, 0.000000000000000000, 1.000000000000000000 ) ) ;
#17099=LINE ( 'NONE', #14611, #28850 ) ;
#17137=FACE_OUTER_BOUND ( 'NONE', #20526, .T. ) ;
#17148=UNCERTAINTY_MEASURE_WITH_UNIT (LENGTH_MEASURE( 1.000000000000000082E-05 ), #21935, 'distance_accuracy_value', 'NONE');
#17150=CYLINDRICAL_SURFACE ( 'NONE', #22805, 1.999999999999999112 ) ;
#17177=CARTESIAN_POINT ( 'NONE',  ( -6.500000000000000000, 0.000000000000000000, 0.000000000000000000 ) ) ;
#17266=DIRECTION ( 'NONE',  ( 0.000000000000000000, 0.000000000000000000, 1.000000000000000000 ) ) ;
#17271=CARTESIAN_POINT ( 'NONE',  ( -6.500000000000000000, 0.000000000000000000, -0.7500000000000000000 ) ) ;
#17353=ORIENTED_EDGE ( 'NONE', *, *, #3680, .F. ) ;
#17360=DIRECTION ( 'NONE',  ( -0.000000000000000000, -0.000000000000000000, 1.000000000000000000 ) ) ;
#17438=DIRECTION ( 'NONE',  ( 0.000000000000000000, 0.000000000000000000, 1.000000000000000000 ) ) ;
#17558=AXIS2_PLACEMENT_3D ( 'NONE', #18697, #29539, #5132 ) ;
#17567=AXIS2_PLACEMENT_3D ( 'NONE', #24365, #19231, #30074 ) ;
#17571=DIRECTION ( 'NONE',  ( 0.000000000000000000, 0.000000000000000000, -1.000000000000000000 ) ) ;
#17585=CIRCLE ( 'NONE', #6750, 1.155000000000000027 ) ;
#17674=DIRECTION ( 'NONE',  ( 1.000000000000000000, 0.000000000000000000, 0.000000000000000000 ) ) ;
#17696=DIRECTION ( 'NONE',  ( 1.000000000000000000, 0.000000000000000000, 0.000000000000000000 ) ) ;
#17716=ORIENTED_EDGE ( 'NONE', *, *, #2145, .T. ) ;
#17753=AXIS2_PLACEMENT_3D ( 'NONE', #31463, #23965, #24141 ) ;
#17768=EDGE_CURVE ( 'NONE', #25058, #26696, #279, .T. ) ;
#17854=( NAMED_UNIT ( * ) PLANE_ANGLE_UNIT ( ) SI_UNIT ( $, .RADIAN. ) );
#17873=FACE_OUTER_BOUND ( 'NONE', #15357, .T. ) ;
#17884=DIRECTION ( 'NONE',  ( -1.000000000000000000, 0.000000000000000000, 0.000000000000000000 ) ) ;
#17906=EDGE_LOOP ( 'NONE', ( #19348, #33291, #607, #15803, #5431, #994, #28229, #9191, #21012 ) ) ;
#17918=CARTESIAN_POINT ( 'NONE',  ( 0.000000000000000000, 0.000000000000000000, -0.7500000000000000000 ) ) ;
#17931=ORIENTED_EDGE ( 'NONE', *, *, #10774, .T. ) ;
#17946=EDGE_CURVE ( 'NONE', #192, #12145, #16756, .T. ) ;
#17971=DIRECTION ( 'NONE',  ( 0.000000000000000000, 0.000000000000000000, -1.000000000000000000 ) ) ;
#18054=DIRECTION ( 'NONE',  ( 1.000000000000000000, 0.000000000000000000, 0.000000000000000000 ) ) ;
#18057=VERTEX_POINT ( 'NONE', #11453 ) ;
#18068=CARTESIAN_POINT ( 'NONE',  ( -1.030735741678193484, 1.713938105891546826, -0.7500000000000000000 ) ) ;
#18345=ORIENTED_EDGE ( 'NONE', *, *, #10774, .F. ) ;
#18510=ORIENTED_EDGE ( 'NONE', *, *, #9484, .T. ) ;
#18561=VERTEX_POINT ( 'NONE', #14450 ) ;
#18660=DIRECTION ( 'NONE',  ( -0.000000000000000000, -0.000000000000000000, -1.000000000000000000 ) ) ;
#18678=FACE_OUTER_BOUND ( 'NONE', #32444, .T. ) ;
#18690=DIRECTION ( 'NONE',  ( 1.000000000000000000, 0.000000000000000000, 0.000000000000000000 ) ) ;
#18697=CARTESIAN_POINT ( 'NONE',  ( 0.000000000000000000, 0.000000000000000000, 5.429999999999999716 ) ) ;
#18746=CARTESIAN_POINT ( 'NONE',  ( -1.030735741678193262, 1.713938105891546382, 4.679999999999999716 ) ) ;
#18823=AXIS2_PLACEMENT_3D ( 'NONE', #14209, #30390, #669 ) ;
#18884=DIRECTION ( 'NONE',  ( 1.000000000000000000, 0.000000000000000000, 0.000000000000000000 ) ) ;
#18886=CIRCLE ( 'NONE', #22201, 1.999999999999999112 ) ;
#18991=ORIENTED_EDGE ( 'NONE', *, *, #12304, .T. ) ;
#19006=CARTESIAN_POINT ( 'NONE',  ( -3.250000000000000000, 5.404196845913421754, 5.429999999999999716 ) ) ;
#19117=ORIENTED_EDGE ( 'NONE', *, *, #9292, .F. ) ;
#19148=FACE_OUTER_BOUND ( 'NONE', #2446, .T. ) ;
#19231=DIRECTION ( 'NONE',  ( -0.000000000000000000, -0.000000000000000000, 1.000000000000000000 ) ) ;
#19235=DIRECTION ( 'NONE',  ( -1.000000000000000000, 0.000000000000000000, -0.000000000000000000 ) ) ;
#19242=CARTESIAN_POINT ( 'NONE',  ( -1.625000000000000000, -1.866624223957557671, 4.679999999999999716 ) ) ;
#19252=ORIENTED_EDGE ( 'NONE', *, *, #12304, .F. ) ;
#19346=VERTEX_POINT ( 'NONE', #25328 ) ;
#19348=ORIENTED_EDGE ( 'NONE', *, *, #16488, .T. ) ;
#19386=EDGE_CURVE ( 'NONE', #20322, #27420, #27050, .T. ) ;
#19388=EDGE_CURVE ( 'NONE', #9166, #18057, #4877, .T. ) ;
#19425=ORIENTED_EDGE ( 'NONE', *, *, #4788, .T. ) ;
#19441=ADVANCED_FACE ( 'NONE', ( #17873 ), #26197, .T. ) ;
#19487=ORIENTED_EDGE ( 'NONE', *, *, #19388, .F. ) ;
#19554=PRODUCT_DEFINITION_FORMATION_WITH_SPECIFIED_SOURCE ( 'ANY', '', #11202, .NOT_KNOWN. ) ;
#19610=VERTEX_POINT ( 'NONE', #18746 ) ;
#19618=DIRECTION ( 'NONE',  ( -1.000000000000000000, 0.000000000000000000, 0.000000000000000000 ) ) ;
#19622=EDGE_CURVE ( 'NONE', #29522, #1801, #25367, .T. ) ;
#19628=DIRECTION ( 'NONE',  ( 0.000000000000000000, 1.000000000000000000, -0.000000000000000000 ) ) ;
#19800=AXIS2_PLACEMENT_3D ( 'NONE', #30820, #3575, #11795 ) ;
#19810=AXIS2_PLACEMENT_3D ( 'NONE', #17271, #25424, #11921 ) ;
#19816=CARTESIAN_POINT ( 'NONE',  ( -4.875000000000000000, -1.866624223957557671, 0.000000000000000000 ) ) ;
#19828=EDGE_LOOP ( 'NONE', ( #14804, #15997, #23011, #6183 ) ) ;
#19963=AXIS2_PLACEMENT_3D ( 'NONE', #27314, #14657, #1457 ) ;
#19980=FACE_OUTER_BOUND ( 'NONE', #4248, .T. ) ;
#20095=AXIS2_PLACEMENT_3D ( 'NONE', #4320, #15206, #1664 ) ;
#20182=EDGE_LOOP ( 'NONE', ( #15017, #19425, #7677, #32188 ) ) ;
#20198=CYLINDRICAL_SURFACE ( 'NONE', #1096, 4.682234377621698584 ) ;
#20204=EDGE_CURVE ( 'NONE', #1801, #4360, #3000, .T. ) ;
#20213=VECTOR ( 'NONE', #10603, 1000.000000000000000 ) ;
#20312=DIRECTION ( 'NONE',  ( 0.000000000000000000, 0.000000000000000000, -1.000000000000000000 ) ) ;
#20322=VERTEX_POINT ( 'NONE', #14595 ) ;
#20398=DIRECTION ( 'NONE',  ( -0.000000000000000000, -0.000000000000000000, 1.000000000000000000 ) ) ;
#20412=CARTESIAN_POINT ( 'NONE',  ( -6.500000000000000000, 0.000000000000000000, -0.7500000000000000000 ) ) ;
#20415=DIRECTION ( 'NONE',  ( -0.000000000000000000, -0.000000000000000000, 1.000000000000000000 ) ) ;
#20517=FACE_OUTER_BOUND ( 'NONE', #17906, .T. ) ;
#20523=DIRECTION ( 'NONE',  ( -0.000000000000000000, -0.000000000000000000, -1.000000000000000000 ) ) ;
#20526=EDGE_LOOP ( 'NONE', ( #1906, #24159, #28632, #14837 ) ) ;
#20538=DIRECTION ( 'NONE',  ( -0.000000000000000000, -0.000000000000000000, 1.000000000000000000 ) ) ;
#20644=ORIENTED_EDGE ( 'NONE', *, *, #32845, .F. ) ;
#20677=EDGE_CURVE ( 'NONE', #4360, #30105, #27526, .T. ) ;
#20697=PLANE ( 'NONE',  #11454 ) ;
#20764=ORIENTED_EDGE ( 'NONE', *, *, #10486, .F. ) ;
#20803=AXIS2_PLACEMENT_3D ( 'NONE', #31205, #4475, #12347 ) ;
#20895=VERTEX_POINT ( 'NONE', #10368 ) ;
#21012=ORIENTED_EDGE ( 'NONE', *, *, #9292, .T. ) ;
#21046=ORIENTED_EDGE ( 'NONE', *, *, #28223, .T. ) ;
#21053=CIRCLE ( 'NONE', #25601, 1.154999999999999805 ) ;
#21054=FACE_BOUND ( 'NONE', #31197, .T. ) ;
#21094=CARTESIAN_POINT ( 'NONE',  ( -0.9727285265192152641, -1.747512292859696670, -0.7500000000000000000 ) ) ;
#21141=CARTESIAN_POINT ( 'NONE',  ( -1.155000000000000027, 0.000000000000000000, 4.679999999999999716 ) ) ;
#21167=CARTESIAN_POINT ( 'NONE',  ( -1.030735741678193262, 1.713938105891546382, 5.429999999999999716 ) ) ;
#21233=DIRECTION ( 'NONE',  ( -1.000000000000000000, 0.000000000000000000, 0.000000000000000000 ) ) ;
#21351=DIRECTION ( 'NONE',  ( -0.000000000000000000, -0.000000000000000000, 1.000000000000000000 ) ) ;
#21352=LINE ( 'NONE', #21167, #11634 ) ;
#21361=DIRECTION ( 'NONE',  ( 0.000000000000000000, 0.000000000000000000, -1.000000000000000000 ) ) ;
#21387=PRODUCT_DEFINITION_CONTEXT ( 'detailed design', #4841, 'design' ) ;
#21422=PRODUCT_DEFINITION ( 'UNKNOWN', '', #19554, #21387 ) ;
#21470=ADVANCED_FACE ( 'NONE', ( #17137 ), #33316, .T. ) ;
#21507=FACE_BOUND ( 'NONE', #25855, .T. ) ;
#21583=PLANE ( 'NONE',  #3752 ) ;
#21609=ADVANCED_FACE ( 'NONE', ( #2140 ), #4272, .F. ) ;
#21730=SHAPE_DEFINITION_REPRESENTATION ( #14933, #15767 ) ;
#21755=CARTESIAN_POINT ( 'NONE',  ( 0.000000000000000000, 0.000000000000000000, -0.7500000000000000000 ) ) ;
#21762=ADVANCED_FACE ( 'NONE', ( #29906 ), #16037, .T. ) ;
#21840=AXIS2_PLACEMENT_3D ( 'NONE', #1433, #20312, #28318 ) ;
#21935=( LENGTH_UNIT ( ) NAMED_UNIT ( * ) SI_UNIT ( .MILLI., .METRE. ) );
#21939=AXIS2_PLACEMENT_3D ( 'NONE', #17918, #12222, #23071 ) ;
#21958=EDGE_LOOP ( 'NONE', ( #6062, #25500, #21046, #15016 ) ) ;
#22005=LINE ( 'NONE', #5962, #14182 ) ;
#22120=CARTESIAN_POINT ( 'NONE',  ( -0.7181323043387221050, -1.866624223957557893, -0.7500000000000000000 ) ) ;
#22125=DIRECTION ( 'NONE',  ( 1.000000000000000000, 0.000000000000000000, 0.000000000000000000 ) ) ;
#22201=AXIS2_PLACEMENT_3D ( 'NONE', #7067, #17971, #34665 ) ;
#22218=EDGE_CURVE ( 'NONE', #14482, #22312, #33359, .T. ) ;
#22219=DIRECTION ( 'NONE',  ( 1.000000000000000000, 0.000000000000000000, 0.000000000000000000 ) ) ;
#22240=ORIENTED_EDGE ( 'NONE', *, *, #10700, .T. ) ;
#22273=CYLINDRICAL_SURFACE ( 'NONE', #3645, 1.154999999999999805 ) ;
#22312=VERTEX_POINT ( 'NONE', #22864 ) ;
#22325=CARTESIAN_POINT ( 'NONE',  ( 1.155000000000000027, 1.414467053015192657E-16, 4.679999999999999716 ) ) ;
#22427=CIRCLE ( 'NONE', #15595, 1.999999999999999556 ) ;
#22435=AXIS2_PLACEMENT_3D ( 'NONE', #12553, #11865, #33732 ) ;
#22452=DIRECTION ( 'NONE',  ( 0.000000000000000000, 0.000000000000000000, -1.000000000000000000 ) ) ;
#22472=CARTESIAN_POINT ( 'NONE',  ( 2.630124765083918348, -1.866624223957557893, -0.7500000000000000000 ) ) ;
#22481=MANIFOLD_SOLID_BREP ( 'Cut-Extrude1', #11099 ) ;
#22589=DIRECTION ( 'NONE',  ( 0.000000000000000000, -0.000000000000000000, 1.000000000000000000 ) ) ;
#22619=ORIENTED_EDGE ( 'NONE', *, *, #382, .T. ) ;
#22633=VECTOR ( 'NONE', #16998, 1000.000000000000000 ) ;
#22698=VECTOR ( 'NONE', #20398, 1000.000000000000000 ) ;
#22709=VERTEX_POINT ( 'NONE', #29016 ) ;
#22805=AXIS2_PLACEMENT_3D ( 'NONE', #3586, #4105, #25831 ) ;
#22842=CARTESIAN_POINT ( 'NONE',  ( 1.999999999999999556, 0.000000000000000000, -0.7500000000000000000 ) ) ;
#22864=CARTESIAN_POINT ( 'NONE',  ( -5.469264258321805627, 1.713938105891546382, 4.679999999999999716 ) ) ;
#22899=CARTESIAN_POINT ( 'NONE',  ( 0.000000000000000000, 0.000000000000000000, 0.000000000000000000 ) ) ;
#22953=CARTESIAN_POINT ( 'NONE',  ( -1.625000000000000000, -1.866624223957557671, 4.679999999999999716 ) ) ;
#23011=ORIENTED_EDGE ( 'NONE', *, *, #4252, .F. ) ;
#23071=DIRECTION ( 'NONE',  ( -1.000000000000000000, 0.000000000000000000, 0.000000000000000000 ) ) ;
#23195=EDGE_LOOP ( 'NONE', ( #28393, #4084, #5210, #6484 ) ) ;
#23252=AXIS2_PLACEMENT_3D ( 'NONE', #33249, #30933, #17438 ) ;
#23256=DIRECTION ( 'NONE',  ( 1.000000000000000000, 0.000000000000000000, 0.000000000000000000 ) ) ;
#23266=DIRECTION ( 'NONE',  ( 1.000000000000000000, 0.000000000000000000, 0.000000000000000000 ) ) ;
#23268=ADVANCED_FACE ( 'NONE', ( #24863 ), #3331, .T. ) ;
#23274=ADVANCED_BREP_SHAPE_REPRESENTATION ( '', ( #22481, #28566 ), #8124 ) ;
#23339=LINE ( 'NONE', #26171, #7051 ) ;
#23360=CARTESIAN_POINT ( 'NONE',  ( 0.000000000000000000, 0.000000000000000000, 0.000000000000000000 ) ) ;
#23373=EDGE_CURVE ( 'NONE', #12065, #14482, #15420, .T. ) ;
#23376=LINE ( 'NONE', #18068, #25250 ) ;
#23417=DIRECTION ( 'NONE',  ( -0.000000000000000000, -0.000000000000000000, -1.000000000000000000 ) ) ;
#23459=LINE ( 'NONE', #21141, #12623 ) ;
#23480=DIRECTION ( 'NONE',  ( -1.000000000000000000, 0.000000000000000000, 0.000000000000000000 ) ) ;
#23537=CARTESIAN_POINT ( 'NONE',  ( -1.030735741678193262, 1.713938105891546382, 5.429999999999999716 ) ) ;
#23553=DIRECTION ( 'NONE',  ( 1.000000000000000000, 0.000000000000000000, 0.000000000000000000 ) ) ;
#23561=CYLINDRICAL_SURFACE ( 'NONE', #6625, 1.155000000000000027 ) ;
#23565=ADVANCED_FACE ( 'NONE', ( #31348 ), #17150, .T. ) ;
#23574=ADVANCED_FACE ( 'NONE', ( #19980 ), #14822, .F. ) ;
#23576=EDGE_CURVE ( 'NONE', #18057, #9166, #4008, .T. ) ;
#23591=ORIENTED_EDGE ( 'NONE', *, *, #15677, .T. ) ;
#23675=ORIENTED_EDGE ( 'NONE', *, *, #8237, .F. ) ;
#23698=ORIENTED_EDGE ( 'NONE', *, *, #28223, .F. ) ;
#23783=VECTOR ( 'NONE', #34935, 1000.000000000000000 ) ;
#23788=CARTESIAN_POINT ( 'NONE',  ( 0.000000000000000000, 0.000000000000000000, 0.000000000000000000 ) ) ;
#23804=ORIENTED_EDGE ( 'NONE', *, *, #8350, .T. ) ;
#23952=VERTEX_POINT ( 'NONE', #1071 ) ;
#23964=AXIS2_PLACEMENT_3D ( 'NONE', #28412, #28585, #6850 ) ;
#23965=DIRECTION ( 'NONE',  ( 0.000000000000000000, 0.000000000000000000, 1.000000000000000000 ) ) ;
#24017=ORIENTED_EDGE ( 'NONE', *, *, #15964, .T. ) ;
#24050=CARTESIAN_POINT ( 'NONE',  ( -0.9727285265192152641, -1.747512292859696670, -0.7500000000000000000 ) ) ;
#24130=VERTEX_POINT ( 'NONE', #2801 ) ;
#24141=DIRECTION ( 'NONE',  ( 1.000000000000000000, 0.000000000000000000, 0.000000000000000000 ) ) ;
#24149=ORIENTED_EDGE ( 'NONE', *, *, #25448, .T. ) ;
#24159=ORIENTED_EDGE ( 'NONE', *, *, #9533, .T. ) ;
#24283=CARTESIAN_POINT ( 'NONE',  ( -7.218132304338721994, -1.866624223957557671, 4.679999999999999716 ) ) ;
#24311=VERTEX_POINT ( 'NONE', #33410 ) ;
#24337=DIRECTION ( 'NONE',  ( 1.000000000000000000, 0.000000000000000000, 0.000000000000000000 ) ) ;
#24365=CARTESIAN_POINT ( 'NONE',  ( -3.250000000000000000, 5.404196845913421754, 0.000000000000000000 ) ) ;
#24381=LINE ( 'NONE', #19242, #32170 ) ;
#24396=LINE ( 'NONE', #2510, #25542 ) ;
#24489=CARTESIAN_POINT ( 'NONE',  ( 1.999999999999999556, 0.000000000000000000, 0.000000000000000000 ) ) ;
#24495=ORIENTED_EDGE ( 'NONE', *, *, #10700, .F. ) ;
#24498=PLANE ( 'NONE',  #32054 ) ;
#24608=DIRECTION ( 'NONE',  ( -0.000000000000000000, -0.000000000000000000, -1.000000000000000000 ) ) ;
#24652=ORIENTED_EDGE ( 'NONE', *, *, #12810, .F. ) ;
#24682=AXIS2_PLACEMENT_3D ( 'NONE', #21755, #34764, #21233 ) ;
#24736=ORIENTED_EDGE ( 'NONE', *, *, #17946, .F. ) ;
#24755=DIRECTION ( 'NONE',  ( 1.000000000000000000, 0.000000000000000000, 0.000000000000000000 ) ) ;
#24863=FACE_OUTER_BOUND ( 'NONE', #9509, .T. ) ;
#24950=ORIENTED_EDGE ( 'NONE', *, *, #4561, .T. ) ;
#24955=ORIENTED_EDGE ( 'NONE', *, *, #12426, .T. ) ;
#25029=CIRCLE ( 'NONE', #23964, 4.306175033202026547 ) ;
#25058=VERTEX_POINT ( 'NONE', #33400 ) ;
#25177=ORIENTED_EDGE ( 'NONE', *, *, #19622, .F. ) ;
#25183=ADVANCED_FACE ( 'NONE', ( #14905 ), #25384, .T. ) ;
#25206=DIRECTION ( 'NONE',  ( 1.000000000000000000, 0.000000000000000000, 0.000000000000000000 ) ) ;
#25229=CARTESIAN_POINT ( 'NONE',  ( -6.500000000000000000, 0.000000000000000000, 0.000000000000000000 ) ) ;
#25250=VECTOR ( 'NONE', #20538, 1000.000000000000000 ) ;
#25328=CARTESIAN_POINT ( 'NONE',  ( -0.7181323043387224381, -1.866624223957557671, 4.679999999999999716 ) ) ;
#25367=CIRCLE ( 'NONE', #31075, 1.999999999999999112 ) ;
#25384=CYLINDRICAL_SURFACE ( 'NONE', #161, 1.999999999999999556 ) ;
#25424=DIRECTION ( 'NONE',  ( 0.000000000000000000, 0.000000000000000000, -1.000000000000000000 ) ) ;
#25433=DIRECTION ( 'NONE',  ( -0.000000000000000000, -0.000000000000000000, 1.000000000000000000 ) ) ;
#25448=EDGE_CURVE ( 'NONE', #22312, #33375, #27464, .T. ) ;
#25489=VERTEX_POINT ( 'NONE', #11481 ) ;
#25500=ORIENTED_EDGE ( 'NONE', *, *, #29938, .T. ) ;
#25532=CIRCLE ( 'NONE', #32923, 1.155000000000000027 ) ;
#25542=VECTOR ( 'NONE', #10887, 1000.000000000000000 ) ;
#25556=DIRECTION ( 'NONE',  ( 0.000000000000000000, 0.000000000000000000, 1.000000000000000000 ) ) ;
#25601=AXIS2_PLACEMENT_3D ( 'NONE', #32322, #2601, #8298 ) ;
#25625=ORIENTED_EDGE ( 'NONE', *, *, #5206, .F. ) ;
#25660=ADVANCED_FACE ( 'NONE', ( #21054, #15738, #31896 ), #13060, .F. ) ;
#25676=DIRECTION ( 'NONE',  ( 1.000000000000000000, 0.000000000000000000, -0.000000000000000000 ) ) ;
#25831=DIRECTION ( 'NONE',  ( -1.000000000000000000, 0.000000000000000000, 0.000000000000000000 ) ) ;
#25839=AXIS2_PLACEMENT_3D ( 'NONE', #1326, #9514, #23553 ) ;
#25855=EDGE_LOOP ( 'NONE', ( #8549, #28096 ) ) ;
#25972=ORIENTED_EDGE ( 'NONE', *, *, #9533, .F. ) ;
#26053=CIRCLE ( 'NONE', #1062, 1.999999999999999556 ) ;
#26171=CARTESIAN_POINT ( 'NONE',  ( -5.527271473480783293, -1.747512292859696226, -0.7500000000000000000 ) ) ;
#26197=CYLINDRICAL_SURFACE ( 'NONE', #20803, 1.999999999999999112 ) ;
#26329=ORIENTED_EDGE ( 'NONE', *, *, #32646, .T. ) ;
#26382=DIRECTION ( 'NONE',  ( -1.000000000000000000, 0.000000000000000000, 0.000000000000000000 ) ) ;
#26444=AXIS2_PLACEMENT_3D ( 'NONE', #29852, #18660, #15820 ) ;
#26450=AXIS2_PLACEMENT_3D ( 'NONE', #2373, #15395, #13254 ) ;
#26558=DIRECTION ( 'NONE',  ( -0.000000000000000000, -0.000000000000000000, -1.000000000000000000 ) ) ;
#26579=CARTESIAN_POINT ( 'NONE',  ( 0.000000000000000000, 0.000000000000000000, 0.000000000000000000 ) ) ;
#26582=ADVANCED_FACE ( 'NONE', ( #21507, #8812, #18678 ), #24498, .F. ) ;
#26606=ORIENTED_EDGE ( 'NONE', *, *, #1635, .F. ) ;
#26612=ORIENTED_EDGE ( 'NONE', *, *, #1889, .F. ) ;
#26626=ORIENTED_EDGE ( 'NONE', *, *, #33988, .T. ) ;
#26656=DIRECTION ( 'NONE',  ( -0.000000000000000000, -0.000000000000000000, -1.000000000000000000 ) ) ;
#26678=CYLINDRICAL_SURFACE ( 'NONE', #10748, 1.999999999999999112 ) ;
#26696=VERTEX_POINT ( 'NONE', #981 ) ;
#26713=ORIENTED_EDGE ( 'NONE', *, *, #3202, .T. ) ;
#26762=DIRECTION ( 'NONE',  ( 0.000000000000000000, 0.000000000000000000, 1.000000000000000000 ) ) ;
#26784=CARTESIAN_POINT ( 'NONE',  ( -5.344999999999999751, 0.000000000000000000, 0.000000000000000000 ) ) ;
#26902=ORIENTED_EDGE ( 'NONE', *, *, #29938, .F. ) ;
#27050=CIRCLE ( 'NONE', #13418, 1.999999999999999556 ) ;
#27169=FACE_OUTER_BOUND ( 'NONE', #34823, .T. ) ;
#27200=DIRECTION ( 'NONE',  ( 0.000000000000000000, 0.000000000000000000, 1.000000000000000000 ) ) ;
#27308=VECTOR ( 'NONE', #4043, 1000.000000000000000 ) ;
#27314=CARTESIAN_POINT ( 'NONE',  ( -3.250000000000000000, -5.838643359331793015, -0.7500000000000000000 ) ) ;
#27420=VERTEX_POINT ( 'NONE', #13374 ) ;
#27437=LINE ( 'NONE', #13571, #5648 ) ;
#27464=CIRCLE ( 'NONE', #33724, 1.999999999999999112 ) ;
#27526=LINE ( 'NONE', #7953, #29968 ) ;
#27564=DIRECTION ( 'NONE',  ( 1.000000000000000000, 0.000000000000000000, 0.000000000000000000 ) ) ;
#27571=ORIENTED_EDGE ( 'NONE', *, *, #25448, .F. ) ;
#27626=CIRCLE ( 'NONE', #21939, 1.999999999999999556 ) ;
#27650=ORIENTED_EDGE ( 'NONE', *, *, #16488, .F. ) ;
#27735=ORIENTED_EDGE ( 'NONE', *, *, #32646, .F. ) ;
#27809=ORIENTED_EDGE ( 'NONE', *, *, #5206, .T. ) ;
#27816=CARTESIAN_POINT ( 'NONE',  ( -3.250000000000000000, -5.838643359331793015, 4.679999999999999716 ) ) ;
#27880=CARTESIAN_POINT ( 'NONE',  ( 0.000000000000000000, 0.000000000000000000, -0.7500000000000000000 ) ) ;
#27958=CARTESIAN_POINT ( 'NONE',  ( -6.500000000000000000, 0.000000000000000000, -0.7520000000000001128 ) ) ;
#27982=CARTESIAN_POINT ( 'NONE',  ( -6.500000000000000000, 0.000000000000000000, 4.679999999999999716 ) ) ;
#27986=ORIENTED_EDGE ( 'NONE', *, *, #2718, .T. ) ;
#28010=DIRECTION ( 'NONE',  ( 1.000000000000000000, -0.000000000000000000, -0.000000000000000000 ) ) ;
#28075=ORIENTED_EDGE ( 'NONE', *, *, #14777, .T. ) ;
#28096=ORIENTED_EDGE ( 'NONE', *, *, #16383, .F. ) ;
#28185=DIRECTION ( 'NONE',  ( 0.000000000000000000, 0.000000000000000000, -1.000000000000000000 ) ) ;
#28201=AXIS2_PLACEMENT_3D ( 'NONE', #9132, #12180, #17696 ) ;
#28223=EDGE_CURVE ( 'NONE', #6836, #14097, #31902, .T. ) ;
#28229=ORIENTED_EDGE ( 'NONE', *, *, #15594, .T. ) ;
#28318=DIRECTION ( 'NONE',  ( -1.000000000000000000, 0.000000000000000000, 0.000000000000000000 ) ) ;
#28393=ORIENTED_EDGE ( 'NONE', *, *, #12670, .T. ) ;
#28401=AXIS2_PLACEMENT_3D ( 'NONE', #6223, #30635, #8913 ) ;
#28412=CARTESIAN_POINT ( 'NONE',  ( -3.250000000000000000, 5.404196845913421754, 4.679999999999999716 ) ) ;
#28487=CARTESIAN_POINT ( 'NONE',  ( 0.000000000000000000, 0.000000000000000000, -0.7500000000000000000 ) ) ;
#28566=AXIS2_PLACEMENT_3D ( 'NONE', #26579, #2200, #13073 ) ;
#28585=DIRECTION ( 'NONE',  ( -0.000000000000000000, -0.000000000000000000, -1.000000000000000000 ) ) ;
#28616=CARTESIAN_POINT ( 'NONE',  ( -5.469264258321805627, 1.713938105891546382, 5.429999999999999716 ) ) ;
#28622=DIRECTION ( 'NONE',  ( 1.000000000000000000, 0.000000000000000000, 0.000000000000000000 ) ) ;
#28632=ORIENTED_EDGE ( 'NONE', *, *, #19388, .T. ) ;
#28685=ORIENTED_EDGE ( 'NONE', *, *, #14375, .F. ) ;
#28729=DIRECTION ( 'NONE',  ( -1.000000000000000000, 0.000000000000000000, 0.000000000000000000 ) ) ;
#28737=EDGE_CURVE ( 'NONE', #23952, #22709, #3707, .T. ) ;
#28753=VERTEX_POINT ( 'NONE', #14938 ) ;
#28850=VECTOR ( 'NONE', #25433, 1000.000000000000000 ) ;
#28907=ORIENTED_EDGE ( 'NONE', *, *, #19386, .T. ) ;
#28921=ORIENTED_EDGE ( 'NONE', *, *, #32625, .T. ) ;
#29016=CARTESIAN_POINT ( 'NONE',  ( -7.218132304338721994, -1.866624223957557671, 0.000000000000000000 ) ) ;
#29065=AXIS2_PLACEMENT_3D ( 'NONE', #23788, #7930, #10791 ) ;
#29077=CARTESIAN_POINT ( 'NONE',  ( 0.000000000000000000, 0.000000000000000000, 4.679999999999999716 ) ) ;
#29182=APPLICATION_CONTEXT ( 'automotive_design' ) ;
#29220=AXIS2_PLACEMENT_3D ( 'NONE', #31688, #34368, #12849 ) ;
#29252=CIRCLE ( 'NONE', #24682, 1.999999999999999556 ) ;
#29286=VERTEX_POINT ( 'NONE', #4648 ) ;
#29310=ADVANCED_FACE ( 'NONE', ( #5180 ), #33, .T. ) ;
#29381=CIRCLE ( 'NONE', #26450, 4.682234377621698584 ) ;
#29468=ORIENTED_EDGE ( 'NONE', *, *, #30130, .T. ) ;
#29522=VERTEX_POINT ( 'NONE', #740 ) ;
#29539=DIRECTION ( 'NONE',  ( 0.000000000000000000, 0.000000000000000000, 1.000000000000000000 ) ) ;
#29599=ORIENTED_EDGE ( 'NONE', *, *, #17946, .T. ) ;
#29852=CARTESIAN_POINT ( 'NONE',  ( 0.000000000000000000, 0.000000000000000000, 4.679999999999999716 ) ) ;
#29906=FACE_OUTER_BOUND ( 'NONE', #16633, .T. ) ;
#29938=EDGE_CURVE ( 'NONE', #7170, #6836, #10854, .T. ) ;
#29968=VECTOR ( 'NONE', #306, 1000.000000000000000 ) ;
#30074=DIRECTION ( 'NONE',  ( -1.000000000000000000, 0.000000000000000000, 0.000000000000000000 ) ) ;
#30105=VERTEX_POINT ( 'NONE', #5104 ) ;
#30130=EDGE_CURVE ( 'NONE', #32547, #14097, #23459, .T. ) ;
#30151=CARTESIAN_POINT ( 'NONE',  ( 0.000000000000000000, 0.000000000000000000, -0.7500000000000000000 ) ) ;
#30156=AXIS2_PLACEMENT_3D ( 'NONE', #15729, #26558, #26382 ) ;
#30200=CIRCLE ( 'NONE', #16581, 1.999999999999999112 ) ;
#30258=VERTEX_POINT ( 'NONE', #24489 ) ;
#30293=( NAMED_UNIT ( * ) PLANE_ANGLE_UNIT ( ) SI_UNIT ( $, .RADIAN. ) );
#30361=LINE ( 'NONE', #472, #11219 ) ;
#30390=DIRECTION ( 'NONE',  ( -0.000000000000000000, -0.000000000000000000, -1.000000000000000000 ) ) ;
#30415=AXIS2_PLACEMENT_3D ( 'NONE', #13537, #13707, #18884 ) ;
#30522=CARTESIAN_POINT ( 'NONE',  ( -5.469264258321805627, 1.713938105891546382, 5.429999999999999716 ) ) ;
#30528=DIRECTION ( 'NONE',  ( 0.000000000000000000, 0.000000000000000000, -1.000000000000000000 ) ) ;
#30622=VERTEX_POINT ( 'NONE', #26784 ) ;
#30635=DIRECTION ( 'NONE',  ( -0.000000000000000000, -0.000000000000000000, 1.000000000000000000 ) ) ;
#30686=LINE ( 'NONE', #6276, #8594 ) ;
#30763=CIRCLE ( 'NONE', #31859, 1.999999999999999556 ) ;
#30820=CARTESIAN_POINT ( 'NONE',  ( -6.500000000000000000, 0.000000000000000000, -0.7520000000000001128 ) ) ;
#30933=DIRECTION ( 'NONE',  ( 0.000000000000000000, 1.000000000000000000, -0.000000000000000000 ) ) ;
#31066=ORIENTED_EDGE ( 'NONE', *, *, #17006, .T. ) ;
#31075=AXIS2_PLACEMENT_3D ( 'NONE', #10191, #12877, #34574 ) ;
#31197=EDGE_LOOP ( 'NONE', ( #2943, #19487 ) ) ;
#31205=CARTESIAN_POINT ( 'NONE',  ( -6.500000000000000000, 0.000000000000000000, 5.429999999999999716 ) ) ;
#31348=FACE_OUTER_BOUND ( 'NONE', #11416, .T. ) ;
#31360=FACE_OUTER_BOUND ( 'NONE', #13954, .T. ) ;
#31405=AXIS2_PLACEMENT_3D ( 'NONE', #4327, #4153, #12899 ) ;
#31428=FACE_OUTER_BOUND ( 'NONE', #3421, .T. ) ;
#31437=DIRECTION ( 'NONE',  ( -0.000000000000000000, -0.000000000000000000, -1.000000000000000000 ) ) ;
#31442=VECTOR ( 'NONE', #6821, 1000.000000000000000 ) ;
#31463=CARTESIAN_POINT ( 'NONE',  ( 0.000000000000000000, 0.000000000000000000, 4.679999999999999716 ) ) ;
#31532=PLANE ( 'NONE',  #14784 ) ;
#31541=CARTESIAN_POINT ( 'NONE',  ( -1.625000000000000000, 2.702098422956710877, 5.429999999999999716 ) ) ;
#31688=CARTESIAN_POINT ( 'NONE',  ( 0.000000000000000000, 0.000000000000000000, 4.679999999999999716 ) ) ;
#31718=CARTESIAN_POINT ( 'NONE',  ( 0.000000000000000000, 0.000000000000000000, 4.679999999999999716 ) ) ;
#31854=CARTESIAN_POINT ( 'NONE',  ( -0.7181323043387221050, -1.866624223957557893, 5.429999999999999716 ) ) ;
#31859=AXIS2_PLACEMENT_3D ( 'NONE', #33385, #17571, #14890 ) ;
#31862=VERTEX_POINT ( 'NONE', #10424 ) ;
#31896=FACE_OUTER_BOUND ( 'NONE', #33906, .T. ) ;
#31902=CIRCLE ( 'NONE', #29065, 1.155000000000000027 ) ;
#31995=DIRECTION ( 'NONE',  ( -1.000000000000000000, 0.000000000000000000, -0.000000000000000000 ) ) ;
#32001=VERTEX_POINT ( 'NONE', #24283 ) ;
#32054=AXIS2_PLACEMENT_3D ( 'NONE', #10826, #30528, #31995 ) ;
#32164=FACE_OUTER_BOUND ( 'NONE', #21958, .T. ) ;
#32170=VECTOR ( 'NONE', #10867, 1000.000000000000000 ) ;
#32188=ORIENTED_EDGE ( 'NONE', *, *, #2145, .F. ) ;
#32273=VECTOR ( 'NONE', #4060, 1000.000000000000000 ) ;
#32322=CARTESIAN_POINT ( 'NONE',  ( -6.500000000000000000, 0.000000000000000000, 0.000000000000000000 ) ) ;
#32408=CYLINDRICAL_SURFACE ( 'NONE', #28401, 1.999999999999999556 ) ;
#32444=EDGE_LOOP ( 'NONE', ( #28685, #14427, #5456, #3708, #13645, #33548, #26612, #33777, #25625 ) ) ;
#32469=DIRECTION ( 'NONE',  ( 0.000000000000000000, 0.000000000000000000, 1.000000000000000000 ) ) ;
#32547=VERTEX_POINT ( 'NONE', #8941 ) ;
#32553=VERTEX_POINT ( 'NONE', #11435 ) ;
#32625=EDGE_CURVE ( 'NONE', #7170, #32547, #5905, .T. ) ;
#32646=EDGE_CURVE ( 'NONE', #10891, #3383, #23339, .T. ) ;
#32662=AXIS2_PLACEMENT_3D ( 'NONE', #16731, #22589, #27564 ) ;
#32699=AXIS2_PLACEMENT_3D ( 'NONE', #29077, #26762, #7012 ) ;
#32721=ORIENTED_EDGE ( 'NONE', *, *, #3202, .F. ) ;
#32734=CARTESIAN_POINT ( 'NONE',  ( 1.155000000000000027, 1.414467053015192657E-16, 4.679999999999999716 ) ) ;
#32781=EDGE_CURVE ( 'NONE', #30105, #192, #8792, .T. ) ;
#32802=DIRECTION ( 'NONE',  ( 1.000000000000000000, 0.000000000000000000, 0.000000000000000000 ) ) ;
#32829=DIRECTION ( 'NONE',  ( -0.000000000000000000, -0.000000000000000000, -1.000000000000000000 ) ) ;
#32845=EDGE_CURVE ( 'NONE', #10974, #10245, #23376, .T. ) ;
#32873=CARTESIAN_POINT ( 'NONE',  ( -8.499999999999998224, 0.000000000000000000, 4.679999999999999716 ) ) ;
#32875=CIRCLE ( 'NONE', #17567, 4.306175033202026547 ) ;
#32923=AXIS2_PLACEMENT_3D ( 'NONE', #31718, #7325, #18054 ) ;
#32963=EDGE_CURVE ( 'NONE', #10974, #20895, #29252, .T. ) ;
#33054=EDGE_CURVE ( 'NONE', #29286, #32553, #14469, .T. ) ;
#33080=CARTESIAN_POINT ( 'NONE',  ( 2.630124765083918348, -1.866624223957557893, 5.429999999999999716 ) ) ;
#33104=CIRCLE ( 'NONE', #31405, 4.306175033202026547 ) ;
#33198=DIRECTION ( 'NONE',  ( 0.000000000000000000, 0.000000000000000000, 1.000000000000000000 ) ) ;
#33249=CARTESIAN_POINT ( 'NONE',  ( 2.630124765083918348, -1.866624223957557893, 5.429999999999999716 ) ) ;
#33290=VECTOR ( 'NONE', #7472, 1000.000000000000000 ) ;
#33291=ORIENTED_EDGE ( 'NONE', *, *, #11136, .T. ) ;
#33316=CYLINDRICAL_SURFACE ( 'NONE', #19800, 1.154999999999999805 ) ;
#33359=LINE ( 'NONE', #30522, #31442 ) ;
#33375=VERTEX_POINT ( 'NONE', #32873 ) ;
#33385=CARTESIAN_POINT ( 'NONE',  ( 0.000000000000000000, 0.000000000000000000, 0.000000000000000000 ) ) ;
#33400=CARTESIAN_POINT ( 'NONE',  ( -5.527271473480783293, -1.747512292859696226, 5.429999999999999716 ) ) ;
#33410=CARTESIAN_POINT ( 'NONE',  ( -5.469264258321805627, 1.713938105891546382, 0.000000000000000000 ) ) ;
#33548=ORIENTED_EDGE ( 'NONE', *, *, #4252, .T. ) ;
#33564=CARTESIAN_POINT ( 'NONE',  ( 1.155000000000000027, 1.414467053015192657E-16, 0.000000000000000000 ) ) ;
#33687=EDGE_LOOP ( 'NONE', ( #23591, #34445, #1552, #26329 ) ) ;
#33724=AXIS2_PLACEMENT_3D ( 'NONE', #16130, #32469, #5415 ) ;
#33732=DIRECTION ( 'NONE',  ( 1.000000000000000000, 0.000000000000000000, 0.000000000000000000 ) ) ;
#33751=DIRECTION ( 'NONE',  ( 1.000000000000000000, 0.000000000000000000, 0.000000000000000000 ) ) ;
#33777=ORIENTED_EDGE ( 'NONE', *, *, #14777, .F. ) ;
#33791=AXIS2_PLACEMENT_3D ( 'NONE', #27816, #24608, #32802 ) ;
#33906=EDGE_LOOP ( 'NONE', ( #26606, #18510, #16131, #24736, #11108, #15201, #8460, #27571, #10656 ) ) ;
#33940=VECTOR ( 'NONE', #16212, 1000.000000000000000 ) ;
#33988=EDGE_CURVE ( 'NONE', #7073, #10974, #33104, .T. ) ;
#33997=CARTESIAN_POINT ( 'NONE',  ( -1.030735741678193484, 1.713938105891546826, -0.7500000000000000000 ) ) ;
#34016=CIRCLE ( 'NONE', #19810, 1.999999999999999112 ) ;
#34074=EDGE_LOOP ( 'NONE', ( #25972, #34143, #14489, #148 ) ) ;
#34085=ORIENTED_EDGE ( 'NONE', *, *, #32845, .T. ) ;
#34143=ORIENTED_EDGE ( 'NONE', *, *, #16383, .T. ) ;
#34184=ORIENTED_EDGE ( 'NONE', *, *, #8237, .T. ) ;
#34210=EDGE_CURVE ( 'NONE', #22709, #24130, #8944, .T. ) ;
#34212=CIRCLE ( 'NONE', #17753, 1.999999999999999556 ) ;
#34219=DIRECTION ( 'NONE',  ( -1.000000000000000000, 0.000000000000000000, 0.000000000000000000 ) ) ;
#34283=ORIENTED_EDGE ( 'NONE', *, *, #33988, .F. ) ;
#34291=STYLED_ITEM('',(#35268),#22481);
#34368=DIRECTION ( 'NONE',  ( 0.000000000000000000, 0.000000000000000000, 1.000000000000000000 ) ) ;
#34445=ORIENTED_EDGE ( 'NONE', *, *, #2562, .T. ) ;
#34507=FACE_OUTER_BOUND ( 'NONE', #2547, .T. ) ;
#34542=LINE ( 'NONE', #31854, #33290 ) ;
#34574=DIRECTION ( 'NONE',  ( 1.000000000000000000, 0.000000000000000000, 0.000000000000000000 ) ) ;
#34613=VECTOR ( 'NONE', #21361, 1000.000000000000000 ) ;
#34665=DIRECTION ( 'NONE',  ( -1.000000000000000000, 0.000000000000000000, 0.000000000000000000 ) ) ;
#34699=CIRCLE ( 'NONE', #9140, 1.999999999999999112 ) ;
#34762=ADVANCED_FACE ( 'NONE', ( #34507 ), #2279, .F. ) ;
#34764=DIRECTION ( 'NONE',  ( 0.000000000000000000, 0.000000000000000000, -1.000000000000000000 ) ) ;
#34823=EDGE_LOOP ( 'NONE', ( #24017, #526, #6499, #17716 ) ) ;
#34935=DIRECTION ( 'NONE',  ( -0.000000000000000000, -0.000000000000000000, 1.000000000000000000 ) ) ;
#34983=CARTESIAN_POINT ( 'NONE',  ( -4.875000000000000000, -1.866624223957557671, 0.000000000000000000 ) ) ;
#35093=SHAPE_REPRESENTATION_RELATIONSHIP ( 'NONE' , 'NONE' ,  #15767, #23274 ) ;
#35262=COLOUR_RGB('Sky Blue',0.24,0.69,0.87);
#35263=FILL_AREA_STYLE_COLOUR('',#35262);
#35264=FILL_AREA_STYLE('',(#35263));
#35265=SURFACE_STYLE_FILL_AREA(#35264);
#35266=SURFACE_SIDE_STYLE('',(#35265));
#35267=SURFACE_STYLE_USAGE(.BOTH.,#35266);
#35268=PRESENTATION_STYLE_ASSIGNMENT((#35267));
ENDSEC;
END-ISO-10303-21;
